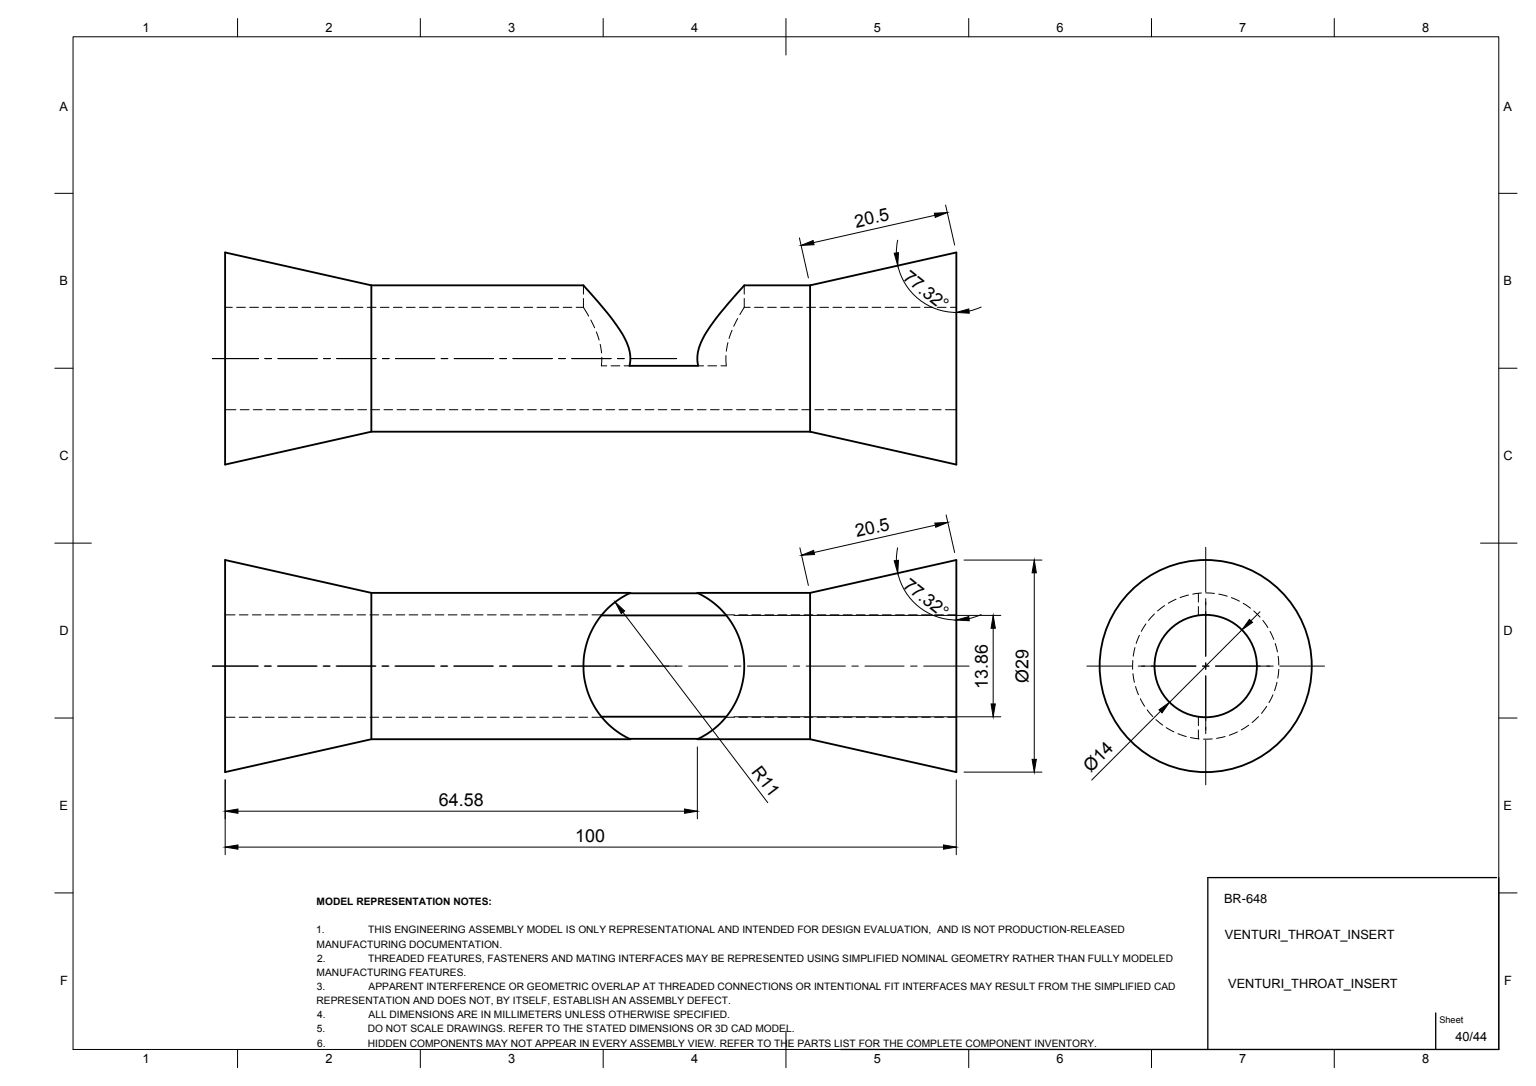
ISO-10303-21;
HEADER;
FILE_DESCRIPTION((''),'2;1');
FILE_NAME('VENTURI_THROAT_INSERT.step','2026-10-01T22:05:39-07:00',(''),(''),'','','');
FILE_SCHEMA (('AUTOMOTIVE_DESIGN { 1 0 10303 214 3 1 1 }'));
ENDSEC;
DATA;
#10=MECHANICAL_DESIGN_GEOMETRIC_PRESENTATION_REPRESENTATION('',(#636),#24628);
#11=CONICAL_SURFACE('',#15204,1.225,0.221314442347791) ;
#12=CONICAL_SURFACE('',#15210,1.225,0.221314442347791) ;
#552=SHAPE_REPRESENTATION_RELATIONSHIP('SRR','None',#24826,#594) ;
#594=ADVANCED_BREP_SHAPE_REPRESENTATION('',(#675),#24616) ;
#636=STYLED_ITEM('',(#25035),#675) ;
#675=MANIFOLD_SOLID_BREP('VENTURI_THROAT_INSERT',#13178) ;
#910=FACE_BOUND('',#4625,.T.) ;
#911=FACE_BOUND('',#4629,.T.) ;
#991=B_SPLINE_CURVE_WITH_KNOTS('',3,(#23937,#23938,#23939,#23940,#23941,
#23942,#23943,#23944,#23945,#23946,#23947,#23948,#23949),.UNSPECIFIED.,
 .F.,.F.,(4,3,2,2,2,4),(-0.0993179449412329,0.,0.274566149486996,0.549132298973992,
0.821321935999811,1.09351157302563),.UNSPECIFIED.) ;
#992=B_SPLINE_CURVE_WITH_KNOTS('',3,(#23951,#23952,#23953,#23954,#23955,
#23956,#23957,#23958,#23959,#23960,#23961,#23962,#23963,#23964,#23965,#23966,
#23967),.UNSPECIFIED.,.F.,.F.,(4,2,2,2,2,2,3,4),(-1.69011593432845,-1.48746936798106,
-1.28482280163367,-0.87952966893888,-0.43976483446944,-0.219882417234721,
0.,0.10342060321835),.UNSPECIFIED.) ;
#993=B_SPLINE_CURVE_WITH_KNOTS('',3,(#23969,#23970,#23971,#23972,#23973,
#23974,#23975,#23976,#23977,#23978,#23979,#23980,#23981,#23982,#23983,#23984),
 .UNSPECIFIED.,.F.,.F.,(4,2,2,2,2,2,2,4),(-3.48365246791255,-3.38023186865691,
-3.16034945142219,-2.94046703418747,-2.50070219971803,-2.09540906702324,
-1.89276250067585,-1.69011593432845),.UNSPECIFIED.) ;
#994=B_SPLINE_CURVE_WITH_KNOTS('',3,(#23987,#23988,#23989,#23990,#23991,
#23992,#23993,#23994,#23995,#23996,#23997,#23998),.UNSPECIFIED.,.F.,.F.,
(4,2,2,2,2,4),(1.09351157302563,1.36570121005145,1.63789084707727,1.91245699656426,
2.18702314605126,2.28634110246251),.UNSPECIFIED.) ;
#995=B_SPLINE_CURVE_WITH_KNOTS('',3,(#24002,#24003,#24004,#24005,#24006,
#24007,#24008,#24009,#24010,#24011,#24012,#24013),.UNSPECIFIED.,.F.,.F.,
(4,2,2,2,2,4),(-2.28634109099249,-2.18702314605126,-1.91245699656426,-1.63789084707727,
-1.36570121005145,-1.09351157302563),.UNSPECIFIED.) ;
#996=B_SPLINE_CURVE_WITH_KNOTS('',3,(#24017,#24018,#24019,#24020,#24021,
#24022,#24023,#24024,#24025,#24026,#24027,#24028,#24029,#24030,#24031,#24032),
 .UNSPECIFIED.,.F.,.F.,(4,2,2,2,2,2,2,4),(1.69011593432845,1.89276250067585,
2.09540906702324,2.50070219971803,2.94046703418747,3.16034945142219,3.38023186865691,
3.48365247187527),.UNSPECIFIED.) ;
#997=B_SPLINE_CURVE_WITH_KNOTS('',3,(#24033,#24034,#24035,#24036,#24037,
#24038,#24039,#24040,#24041,#24042,#24043,#24044,#24045,#24046,#24047,#24048,
#24049),.UNSPECIFIED.,.F.,.F.,(4,3,2,2,2,2,2,4),(-0.103420599255634,0.,
0.21988241723472,0.43976483446944,0.87952966893888,1.28482280163367,1.48746936798106,
1.69011593432845),.UNSPECIFIED.) ;
#998=B_SPLINE_CURVE_WITH_KNOTS('',3,(#24050,#24051,#24052,#24053,#24054,
#24055,#24056,#24057,#24058,#24059,#24060,#24061,#24062),.UNSPECIFIED.,
 .F.,.F.,(4,2,2,2,3,4),(-1.09351157302563,-0.821321935999811,-0.549132298973992,
-0.274566149486996,0.,0.0993179564112534),.UNSPECIFIED.) ;
#1712=LINE('',#23929,#2548) ;
#1713=LINE('',#23933,#2549) ;
#1714=LINE('',#24064,#2550) ;
#1715=LINE('',#24065,#2551) ;
#1716=LINE('',#24069,#2552) ;
#1717=LINE('',#24071,#2553) ;
#1718=LINE('',#24077,#2554) ;
#1719=LINE('',#24081,#2555) ;
#1720=LINE('',#24083,#2556) ;
#1721=LINE('',#24087,#2557) ;
#2548=VECTOR('',#19185,1.) ;
#2549=VECTOR('',#19188,1.) ;
#2550=VECTOR('',#19201,1.) ;
#2551=VECTOR('',#19202,1.) ;
#2552=VECTOR('',#19207,0.7) ;
#2553=VECTOR('',#19208,0.7) ;
#2554=VECTOR('',#19215,1.225) ;
#2555=VECTOR('',#19222,1.) ;
#2556=VECTOR('',#19223,1.) ;
#2557=VECTOR('',#19228,1.225) ;
#2920=CYLINDRICAL_SURFACE('',#15196,1.1) ;
#2921=CYLINDRICAL_SURFACE('',#15198,1.1) ;
#2922=CYLINDRICAL_SURFACE('',#15201,0.7) ;
#2923=CYLINDRICAL_SURFACE('',#15208,1.) ;
#3627=FACE_OUTER_BOUND('',#4618,.T.) ;
#3628=FACE_OUTER_BOUND('',#4619,.T.) ;
#3629=FACE_OUTER_BOUND('',#4620,.T.) ;
#3630=FACE_OUTER_BOUND('',#4621,.T.) ;
#3631=FACE_OUTER_BOUND('',#4622,.T.) ;
#3632=FACE_OUTER_BOUND('',#4623,.T.) ;
#3633=FACE_OUTER_BOUND('',#4624,.T.) ;
#3634=FACE_OUTER_BOUND('',#4626,.T.) ;
#3635=FACE_OUTER_BOUND('',#4627,.T.) ;
#3636=FACE_OUTER_BOUND('',#4628,.T.) ;
#4618=EDGE_LOOP('',(#11597,#11598,#11599,#11600)) ;
#4619=EDGE_LOOP('',(#11601,#11602,#11603,#11604,#11605,#11606)) ;
#4620=EDGE_LOOP('',(#11607,#11608,#11609,#11610,#11611,#11612)) ;
#4621=EDGE_LOOP('',(#11613,#11614,#11615,#11616)) ;
#4622=EDGE_LOOP('',(#11617,#11618,#11619,#11620,#11621,#11622,#11623,#11624,
#11625,#11626,#11627,#11628)) ;
#4623=EDGE_LOOP('',(#11629,#11630,#11631,#11632)) ;
#4624=EDGE_LOOP('',(#11633)) ;
#4625=EDGE_LOOP('',(#11634)) ;
#4626=EDGE_LOOP('',(#11635,#11636,#11637,#11638,#11639,#11640,#11641,#11642,
#11643,#11644,#11645,#11646)) ;
#4627=EDGE_LOOP('',(#11647,#11648,#11649,#11650)) ;
#4628=EDGE_LOOP('',(#11651)) ;
#4629=EDGE_LOOP('',(#11652)) ;
#5473=CIRCLE('',#15194,1.1) ;
#5474=CIRCLE('',#15195,1.1) ;
#5475=CIRCLE('',#15197,1.1) ;
#5476=CIRCLE('',#15199,1.1) ;
#5477=CIRCLE('',#15202,0.7) ;
#5478=CIRCLE('',#15203,0.7) ;
#5479=CIRCLE('',#15205,1.45) ;
#5480=CIRCLE('',#15206,1.) ;
#5481=CIRCLE('',#15209,1.) ;
#5482=CIRCLE('',#15211,1.45) ;
#6601=VERTEX_POINT('',#23927) ;
#6602=VERTEX_POINT('',#23928) ;
#6603=VERTEX_POINT('',#23930) ;
#6604=VERTEX_POINT('',#23932) ;
#6605=VERTEX_POINT('',#23936) ;
#6606=VERTEX_POINT('',#23950) ;
#6607=VERTEX_POINT('',#23968) ;
#6608=VERTEX_POINT('',#23985) ;
#6609=VERTEX_POINT('',#24000) ;
#6610=VERTEX_POINT('',#24001) ;
#6611=VERTEX_POINT('',#24014) ;
#6612=VERTEX_POINT('',#24016) ;
#6613=VERTEX_POINT('',#24067) ;
#6614=VERTEX_POINT('',#24070) ;
#6615=VERTEX_POINT('',#24074) ;
#6616=VERTEX_POINT('',#24076) ;
#6617=VERTEX_POINT('',#24082) ;
#6618=VERTEX_POINT('',#24086) ;
#8288=EDGE_CURVE('',#6601,#6602,#1712,.T.) ;
#8289=EDGE_CURVE('',#6603,#6601,#5473,.T.) ;
#8290=EDGE_CURVE('',#6604,#6603,#1713,.T.) ;
#8291=EDGE_CURVE('',#6602,#6604,#5474,.T.) ;
#8292=EDGE_CURVE('',#6602,#6605,#991,.T.) ;
#8293=EDGE_CURVE('',#6606,#6604,#992,.T.) ;
#8294=EDGE_CURVE('',#6607,#6606,#993,.T.) ;
#8295=EDGE_CURVE('',#6607,#6608,#5475,.T.) ;
#8296=EDGE_CURVE('',#6605,#6608,#994,.T.) ;
#8297=EDGE_CURVE('',#6609,#6610,#995,.T.) ;
#8298=EDGE_CURVE('',#6609,#6611,#5476,.T.) ;
#8299=EDGE_CURVE('',#6612,#6611,#996,.T.) ;
#8300=EDGE_CURVE('',#6603,#6612,#997,.T.) ;
#8301=EDGE_CURVE('',#6610,#6601,#998,.T.) ;
#8302=EDGE_CURVE('',#6608,#6609,#1714,.T.) ;
#8303=EDGE_CURVE('',#6611,#6607,#1715,.T.) ;
#8304=EDGE_CURVE('',#6613,#6613,#5477,.T.) ;
#8305=EDGE_CURVE('',#6613,#6605,#1716,.T.) ;
#8306=EDGE_CURVE('',#6610,#6614,#1717,.T.) ;
#8307=EDGE_CURVE('',#6614,#6614,#5478,.T.) ;
#8308=EDGE_CURVE('',#6615,#6615,#5479,.T.) ;
#8309=EDGE_CURVE('',#6615,#6616,#1718,.T.) ;
#8310=EDGE_CURVE('',#6616,#6616,#5480,.T.) ;
#8311=EDGE_CURVE('',#6616,#6612,#1719,.T.) ;
#8312=EDGE_CURVE('',#6606,#6617,#1720,.T.) ;
#8313=EDGE_CURVE('',#6617,#6617,#5481,.T.) ;
#8314=EDGE_CURVE('',#6617,#6618,#1721,.T.) ;
#8315=EDGE_CURVE('',#6618,#6618,#5482,.T.) ;
#11597=ORIENTED_EDGE('',*,*,#8288,.F.) ;
#11598=ORIENTED_EDGE('',*,*,#8289,.F.) ;
#11599=ORIENTED_EDGE('',*,*,#8290,.F.) ;
#11600=ORIENTED_EDGE('',*,*,#8291,.F.) ;
#11601=ORIENTED_EDGE('',*,*,#8292,.F.) ;
#11602=ORIENTED_EDGE('',*,*,#8291,.T.) ;
#11603=ORIENTED_EDGE('',*,*,#8293,.F.) ;
#11604=ORIENTED_EDGE('',*,*,#8294,.F.) ;
#11605=ORIENTED_EDGE('',*,*,#8295,.T.) ;
#11606=ORIENTED_EDGE('',*,*,#8296,.F.) ;
#11607=ORIENTED_EDGE('',*,*,#8297,.F.) ;
#11608=ORIENTED_EDGE('',*,*,#8298,.T.) ;
#11609=ORIENTED_EDGE('',*,*,#8299,.F.) ;
#11610=ORIENTED_EDGE('',*,*,#8300,.F.) ;
#11611=ORIENTED_EDGE('',*,*,#8289,.T.) ;
#11612=ORIENTED_EDGE('',*,*,#8301,.F.) ;
#11613=ORIENTED_EDGE('',*,*,#8302,.F.) ;
#11614=ORIENTED_EDGE('',*,*,#8295,.F.) ;
#11615=ORIENTED_EDGE('',*,*,#8303,.F.) ;
#11616=ORIENTED_EDGE('',*,*,#8298,.F.) ;
#11617=ORIENTED_EDGE('',*,*,#8304,.F.) ;
#11618=ORIENTED_EDGE('',*,*,#8305,.T.) ;
#11619=ORIENTED_EDGE('',*,*,#8296,.T.) ;
#11620=ORIENTED_EDGE('',*,*,#8302,.T.) ;
#11621=ORIENTED_EDGE('',*,*,#8297,.T.) ;
#11622=ORIENTED_EDGE('',*,*,#8306,.T.) ;
#11623=ORIENTED_EDGE('',*,*,#8307,.F.) ;
#11624=ORIENTED_EDGE('',*,*,#8306,.F.) ;
#11625=ORIENTED_EDGE('',*,*,#8301,.T.) ;
#11626=ORIENTED_EDGE('',*,*,#8288,.T.) ;
#11627=ORIENTED_EDGE('',*,*,#8292,.T.) ;
#11628=ORIENTED_EDGE('',*,*,#8305,.F.) ;
#11629=ORIENTED_EDGE('',*,*,#8308,.F.) ;
#11630=ORIENTED_EDGE('',*,*,#8309,.T.) ;
#11631=ORIENTED_EDGE('',*,*,#8310,.T.) ;
#11632=ORIENTED_EDGE('',*,*,#8309,.F.) ;
#11633=ORIENTED_EDGE('',*,*,#8308,.T.) ;
#11634=ORIENTED_EDGE('',*,*,#8307,.T.) ;
#11635=ORIENTED_EDGE('',*,*,#8310,.F.) ;
#11636=ORIENTED_EDGE('',*,*,#8311,.T.) ;
#11637=ORIENTED_EDGE('',*,*,#8299,.T.) ;
#11638=ORIENTED_EDGE('',*,*,#8303,.T.) ;
#11639=ORIENTED_EDGE('',*,*,#8294,.T.) ;
#11640=ORIENTED_EDGE('',*,*,#8312,.T.) ;
#11641=ORIENTED_EDGE('',*,*,#8313,.T.) ;
#11642=ORIENTED_EDGE('',*,*,#8312,.F.) ;
#11643=ORIENTED_EDGE('',*,*,#8293,.T.) ;
#11644=ORIENTED_EDGE('',*,*,#8290,.T.) ;
#11645=ORIENTED_EDGE('',*,*,#8300,.T.) ;
#11646=ORIENTED_EDGE('',*,*,#8311,.F.) ;
#11647=ORIENTED_EDGE('',*,*,#8313,.F.) ;
#11648=ORIENTED_EDGE('',*,*,#8314,.T.) ;
#11649=ORIENTED_EDGE('',*,*,#8315,.F.) ;
#11650=ORIENTED_EDGE('',*,*,#8314,.F.) ;
#11651=ORIENTED_EDGE('',*,*,#8315,.T.) ;
#11652=ORIENTED_EDGE('',*,*,#8304,.T.) ;
#12289=PLANE('',#15193) ;
#12290=PLANE('',#15200) ;
#12291=PLANE('',#15207) ;
#12292=PLANE('',#15212) ;
#13022=ADVANCED_FACE('',(#3627),#12289,.F.) ;
#13023=ADVANCED_FACE('',(#3628),#2920,.F.) ;
#13024=ADVANCED_FACE('',(#3629),#2921,.F.) ;
#13025=ADVANCED_FACE('',(#3630),#12290,.F.) ;
#13026=ADVANCED_FACE('',(#3631),#2922,.F.) ;
#13027=ADVANCED_FACE('',(#3632),#11,.T.) ;
#13028=ADVANCED_FACE('',(#3633,#910),#12291,.T.) ;
#13029=ADVANCED_FACE('',(#3634),#2923,.T.) ;
#13030=ADVANCED_FACE('',(#3635),#12,.T.) ;
#13031=ADVANCED_FACE('',(#3636,#911),#12292,.T.) ;
#13178=CLOSED_SHELL('',(#13022,#13023,#13024,#13025,#13026,#13027,#13028,
#13029,#13030,#13031)) ;
#15192=AXIS2_PLACEMENT_3D('',#23925,#19181,#19182) ;
#15193=AXIS2_PLACEMENT_3D('',#23926,#19183,#19184) ;
#15194=AXIS2_PLACEMENT_3D('',#23931,#19186,#19187) ;
#15195=AXIS2_PLACEMENT_3D('',#23934,#19189,#19190) ;
#15196=AXIS2_PLACEMENT_3D('',#23935,#19191,#19192) ;
#15197=AXIS2_PLACEMENT_3D('',#23986,#19193,#19194) ;
#15198=AXIS2_PLACEMENT_3D('',#23999,#19195,#19196) ;
#15199=AXIS2_PLACEMENT_3D('',#24015,#19197,#19198) ;
#15200=AXIS2_PLACEMENT_3D('',#24063,#19199,#19200) ;
#15201=AXIS2_PLACEMENT_3D('',#24066,#19203,#19204) ;
#15202=AXIS2_PLACEMENT_3D('',#24068,#19205,#19206) ;
#15203=AXIS2_PLACEMENT_3D('',#24072,#19209,#19210) ;
#15204=AXIS2_PLACEMENT_3D('',#24073,#19211,#19212) ;
#15205=AXIS2_PLACEMENT_3D('',#24075,#19213,#19214) ;
#15206=AXIS2_PLACEMENT_3D('',#24078,#19216,#19217) ;
#15207=AXIS2_PLACEMENT_3D('',#24079,#19218,#19219) ;
#15208=AXIS2_PLACEMENT_3D('',#24080,#19220,#19221) ;
#15209=AXIS2_PLACEMENT_3D('',#24084,#19224,#19225) ;
#15210=AXIS2_PLACEMENT_3D('',#24085,#19226,#19227) ;
#15211=AXIS2_PLACEMENT_3D('',#24088,#19229,#19230) ;
#15212=AXIS2_PLACEMENT_3D('',#24089,#19231,#19232) ;
#19181=DIRECTION('axis',(0.,0.,1.)) ;
#19182=DIRECTION('refdir',(1.,0.,0.)) ;
#19183=DIRECTION('center_axis',(0.,0.,-1.)) ;
#19184=DIRECTION('ref_axis',(-1.,0.,0.)) ;
#19185=DIRECTION('',(-1.,0.,0.)) ;
#19186=DIRECTION('center_axis',(0.,0.,-1.)) ;
#19187=DIRECTION('ref_axis',(1.,0.,0.)) ;
#19188=DIRECTION('',(1.,0.,0.)) ;
#19189=DIRECTION('center_axis',(0.,0.,-1.)) ;
#19190=DIRECTION('ref_axis',(1.,0.,0.)) ;
#19191=DIRECTION('center_axis',(0.,0.,1.)) ;
#19192=DIRECTION('ref_axis',(-1.,-1.22464679914735E-16,0.)) ;
#19193=DIRECTION('center_axis',(0.,0.,-1.)) ;
#19194=DIRECTION('ref_axis',(1.,0.,0.)) ;
#19195=DIRECTION('center_axis',(0.,0.,1.)) ;
#19196=DIRECTION('ref_axis',(1.,0.,0.)) ;
#19197=DIRECTION('center_axis',(0.,0.,-1.)) ;
#19198=DIRECTION('ref_axis',(1.,0.,0.)) ;
#19199=DIRECTION('center_axis',(0.,0.,-1.)) ;
#19200=DIRECTION('ref_axis',(-1.,0.,0.)) ;
#19201=DIRECTION('',(1.,0.,0.)) ;
#19202=DIRECTION('',(-1.,0.,0.)) ;
#19203=DIRECTION('center_axis',(1.,0.,0.)) ;
#19204=DIRECTION('ref_axis',(0.,0.,-1.)) ;
#19205=DIRECTION('center_axis',(1.,0.,0.)) ;
#19206=DIRECTION('ref_axis',(0.,0.,-1.)) ;
#19207=DIRECTION('',(1.,0.,0.)) ;
#19208=DIRECTION('',(1.,0.,0.)) ;
#19209=DIRECTION('center_axis',(-1.,0.,0.)) ;
#19210=DIRECTION('ref_axis',(0.,0.,-1.)) ;
#19211=DIRECTION('center_axis',(1.,0.,0.)) ;
#19212=DIRECTION('ref_axis',(0.,0.,-1.)) ;
#19213=DIRECTION('center_axis',(1.,0.,0.)) ;
#19214=DIRECTION('ref_axis',(0.,0.,-1.)) ;
#19215=DIRECTION('',(-0.975609756097561,2.68824907129907E-17,-0.219512195121951)) ;
#19216=DIRECTION('center_axis',(1.,0.,0.)) ;
#19217=DIRECTION('ref_axis',(0.,0.,-1.)) ;
#19218=DIRECTION('center_axis',(1.,0.,0.)) ;
#19219=DIRECTION('ref_axis',(0.,0.,-1.)) ;
#19220=DIRECTION('center_axis',(1.,0.,0.)) ;
#19221=DIRECTION('ref_axis',(0.,0.,-1.)) ;
#19222=DIRECTION('',(-1.,0.,0.)) ;
#19223=DIRECTION('',(-1.,0.,0.)) ;
#19224=DIRECTION('center_axis',(1.,0.,0.)) ;
#19225=DIRECTION('ref_axis',(0.,0.,-1.)) ;
#19226=DIRECTION('center_axis',(-1.,0.,0.)) ;
#19227=DIRECTION('ref_axis',(0.,0.,-1.)) ;
#19228=DIRECTION('',(-0.975609756097561,-2.68824907129907E-17,0.219512195121951)) ;
#19229=DIRECTION('center_axis',(-1.,0.,0.)) ;
#19230=DIRECTION('ref_axis',(0.,0.,-1.)) ;
#19231=DIRECTION('center_axis',(-1.,0.,0.)) ;
#19232=DIRECTION('ref_axis',(0.,0.,1.)) ;
#23925=CARTESIAN_POINT('',(0.,0.,0.)) ;
#23926=CARTESIAN_POINT('Origin',(-3.,-1.8,-16.6)) ;
#23927=CARTESIAN_POINT('',(-2.14559962546825,-1.10717967697245,-16.6)) ;
#23928=CARTESIAN_POINT('',(-3.85440037453175,-1.10717967697245,-16.6)) ;
#23929=CARTESIAN_POINT('',(-4.,-1.10717967697245,-16.6)) ;
#23930=CARTESIAN_POINT('',(-2.53095842401766,-0.80501256289338,-16.6)) ;
#23931=CARTESIAN_POINT('Origin',(-3.,-1.8,-16.6)) ;
#23932=CARTESIAN_POINT('',(-3.46904157598234,-0.80501256289338,-16.6)) ;
#23933=CARTESIAN_POINT('',(-4.,-0.80501256289338,-16.6)) ;
#23934=CARTESIAN_POINT('Origin',(-3.,-1.8,-16.6)) ;
#23935=CARTESIAN_POINT('Origin',(-3.,-1.8,-15.55)) ;
#23936=CARTESIAN_POINT('',(-4.1,-1.8,-15.8)) ;
#23937=CARTESIAN_POINT('Ctrl Pts',(-3.85440037453175,-1.10717967697245,
-16.6)) ;
#23938=CARTESIAN_POINT('Ctrl Pts',(-3.85049705318298,-1.10236602022558,
-16.5666500077769)) ;
#23939=CARTESIAN_POINT('Ctrl Pts',(-3.84852813742386,-1.1,-16.5331059816471)) ;
#23940=CARTESIAN_POINT('Ctrl Pts',(-3.84852813742386,-1.1,-16.5)) ;
#23941=CARTESIAN_POINT('Ctrl Pts',(-3.84852813742386,-1.1,-16.408477950171)) ;
#23942=CARTESIAN_POINT('Ctrl Pts',(-3.86487430708359,-1.11884674360792,
-16.3138744868034)) ;
#23943=CARTESIAN_POINT('Ctrl Pts',(-3.91703156085527,-1.19087751926739,
-16.1428129676115)) ;
#23944=CARTESIAN_POINT('Ctrl Pts',(-3.95162711030062,-1.24406317485413,
-16.0659873314847)) ;
#23945=CARTESIAN_POINT('Ctrl Pts',(-4.01279528835241,-1.36545967307144,
-15.9445908332674)) ;
#23946=CARTESIAN_POINT('Ctrl Pts',(-4.04402775497001,-1.44241519978942,
-15.8910472783858)) ;
#23947=CARTESIAN_POINT('Ctrl Pts',(-4.08782165352582,-1.6142450358863,-15.8186884461636)) ;
#23948=CARTESIAN_POINT('Ctrl Pts',(-4.1,-1.70927012099139,-15.8)) ;
#23949=CARTESIAN_POINT('Ctrl Pts',(-4.1,-1.8,-15.8)) ;
#23950=CARTESIAN_POINT('',(-4.1,-1.8,-15.5)) ;
#23951=CARTESIAN_POINT('Ctrl Pts',(-4.1,-1.8,-15.5)) ;
#23952=CARTESIAN_POINT('Ctrl Pts',(-4.1,-1.73245114455087,-15.5)) ;
#23953=CARTESIAN_POINT('Ctrl Pts',(-4.09366900622909,-1.66396811523288,
-15.5069510256229)) ;
#23954=CARTESIAN_POINT('Ctrl Pts',(-4.06861417966391,-1.53040715178794,
-15.5346137377671)) ;
#23955=CARTESIAN_POINT('Ctrl Pts',(-4.04990213252851,-1.46532446507313,
-15.5553131496202)) ;
#23956=CARTESIAN_POINT('Ctrl Pts',(-3.97908681363415,-1.28173592783325,
-15.6344562293198)) ;
#23957=CARTESIAN_POINT('Ctrl Pts',(-3.91155673921738,-1.17504680959349,
-15.7107396280334)) ;
#23958=CARTESIAN_POINT('Ctrl Pts',(-3.76780945986836,-1.00375215686099,
-15.8820342807659)) ;
#23959=CARTESIAN_POINT('Ctrl Pts',(-3.67938152899323,-0.930008802100376,
-15.9904145776246)) ;
#23960=CARTESIAN_POINT('Ctrl Pts',(-3.56405332421194,-0.85450777858214,
-16.1680616160286)) ;
#23961=CARTESIAN_POINT('Ctrl Pts',(-3.52879854306256,-0.834982894950926,
-16.2296167208294)) ;
#23962=CARTESIAN_POINT('Ctrl Pts',(-3.47583842827067,-0.807798528642412,
-16.3589280031455)) ;
#23963=CARTESIAN_POINT('Ctrl Pts',(-3.45825756949558,-0.8,-16.4267058609218)) ;
#23964=CARTESIAN_POINT('Ctrl Pts',(-3.45825756949558,-0.8,-16.5)) ;
#23965=CARTESIAN_POINT('Ctrl Pts',(-3.45825756949558,-0.8,-16.5344735344061)) ;
#23966=CARTESIAN_POINT('Ctrl Pts',(-3.46215940235726,-0.801768275133648,
-16.5677197443671)) ;
#23967=CARTESIAN_POINT('Ctrl Pts',(-3.46904157598234,-0.80501256289338,
-16.6)) ;
#23968=CARTESIAN_POINT('',(-3.46904157598234,-2.79498743710662,-16.6)) ;
#23969=CARTESIAN_POINT('Ctrl Pts',(-3.46904157598234,-2.79498743710662,
-16.6)) ;
#23970=CARTESIAN_POINT('Ctrl Pts',(-3.46215940232543,-2.79823172488136,
-16.5677197442178)) ;
#23971=CARTESIAN_POINT('Ctrl Pts',(-3.45825756949559,-2.8,-16.5344735330852)) ;
#23972=CARTESIAN_POINT('Ctrl Pts',(-3.45825756949558,-2.8,-16.4267058609218)) ;
#23973=CARTESIAN_POINT('Ctrl Pts',(-3.47583842827066,-2.79220147135759,
-16.3589280031455)) ;
#23974=CARTESIAN_POINT('Ctrl Pts',(-3.52879854306256,-2.76501710504908,
-16.2296167208294)) ;
#23975=CARTESIAN_POINT('Ctrl Pts',(-3.56405332421193,-2.74549222141786,
-16.1680616160286)) ;
#23976=CARTESIAN_POINT('Ctrl Pts',(-3.67938152899323,-2.66999119789963,
-15.9904145776246)) ;
#23977=CARTESIAN_POINT('Ctrl Pts',(-3.76780945986836,-2.59624784313901,
-15.8820342807659)) ;
#23978=CARTESIAN_POINT('Ctrl Pts',(-3.91155673921738,-2.42495319040651,
-15.7107396280334)) ;
#23979=CARTESIAN_POINT('Ctrl Pts',(-3.97908681363414,-2.31826407216675,
-15.6344562293198)) ;
#23980=CARTESIAN_POINT('Ctrl Pts',(-4.04990213252851,-2.13467553492687,
-15.5553131496202)) ;
#23981=CARTESIAN_POINT('Ctrl Pts',(-4.06861417966391,-2.06959284821206,
-15.5346137377671)) ;
#23982=CARTESIAN_POINT('Ctrl Pts',(-4.09366900622909,-1.93603188476712,
-15.5069510256229)) ;
#23983=CARTESIAN_POINT('Ctrl Pts',(-4.1,-1.86754885544913,-15.5)) ;
#23984=CARTESIAN_POINT('Ctrl Pts',(-4.1,-1.8,-15.5)) ;
#23985=CARTESIAN_POINT('',(-3.85440037453175,-2.49282032302755,-16.6)) ;
#23986=CARTESIAN_POINT('Origin',(-3.,-1.8,-16.6)) ;
#23987=CARTESIAN_POINT('Ctrl Pts',(-4.1,-1.8,-15.8)) ;
#23988=CARTESIAN_POINT('Ctrl Pts',(-4.1,-1.89072987900861,-15.8)) ;
#23989=CARTESIAN_POINT('Ctrl Pts',(-4.08782165352582,-1.9857549641137,-15.8186884461636)) ;
#23990=CARTESIAN_POINT('Ctrl Pts',(-4.04402775497001,-2.15758480021059,
-15.8910472783858)) ;
#23991=CARTESIAN_POINT('Ctrl Pts',(-4.01279528835241,-2.23454032692856,
-15.9445908332674)) ;
#23992=CARTESIAN_POINT('Ctrl Pts',(-3.95162711030062,-2.35593682514587,
-16.0659873314847)) ;
#23993=CARTESIAN_POINT('Ctrl Pts',(-3.91703156085527,-2.40912248073261,
-16.1428129676115)) ;
#23994=CARTESIAN_POINT('Ctrl Pts',(-3.86487430708359,-2.48115325639208,
-16.3138744868034)) ;
#23995=CARTESIAN_POINT('Ctrl Pts',(-3.84852813742386,-2.5,-16.408477950171)) ;
#23996=CARTESIAN_POINT('Ctrl Pts',(-3.84852813742386,-2.5,-16.5331059854704)) ;
#23997=CARTESIAN_POINT('Ctrl Pts',(-3.85049705337729,-2.4976339795348,-16.5666500094371)) ;
#23998=CARTESIAN_POINT('Ctrl Pts',(-3.85440037453175,-2.49282032302755,
-16.6)) ;
#23999=CARTESIAN_POINT('Origin',(-3.,-1.8,-15.55)) ;
#24000=CARTESIAN_POINT('',(-2.14559962546825,-2.49282032302755,-16.6)) ;
#24001=CARTESIAN_POINT('',(-1.9,-1.8,-15.8)) ;
#24002=CARTESIAN_POINT('Ctrl Pts',(-2.14559962546825,-2.49282032302755,
-16.6)) ;
#24003=CARTESIAN_POINT('Ctrl Pts',(-2.14950294681702,-2.49763397977442,
-16.5666500077769)) ;
#24004=CARTESIAN_POINT('Ctrl Pts',(-2.15147186257614,-2.5,-16.5331059816471)) ;
#24005=CARTESIAN_POINT('Ctrl Pts',(-2.15147186257614,-2.5,-16.408477950171)) ;
#24006=CARTESIAN_POINT('Ctrl Pts',(-2.13512569291641,-2.48115325639208,
-16.3138744868034)) ;
#24007=CARTESIAN_POINT('Ctrl Pts',(-2.08296843914473,-2.40912248073261,
-16.1428129676115)) ;
#24008=CARTESIAN_POINT('Ctrl Pts',(-2.04837288969938,-2.35593682514587,
-16.0659873314847)) ;
#24009=CARTESIAN_POINT('Ctrl Pts',(-1.98720471164759,-2.23454032692856,
-15.9445908332674)) ;
#24010=CARTESIAN_POINT('Ctrl Pts',(-1.95597224502999,-2.15758480021059,
-15.8910472783858)) ;
#24011=CARTESIAN_POINT('Ctrl Pts',(-1.91217834647418,-1.9857549641137,-15.8186884461636)) ;
#24012=CARTESIAN_POINT('Ctrl Pts',(-1.9,-1.89072987900861,-15.8)) ;
#24013=CARTESIAN_POINT('Ctrl Pts',(-1.9,-1.8,-15.8)) ;
#24014=CARTESIAN_POINT('',(-2.53095842401766,-2.79498743710662,-16.6)) ;
#24015=CARTESIAN_POINT('Origin',(-3.,-1.8,-16.6)) ;
#24016=CARTESIAN_POINT('',(-1.9,-1.8,-15.5)) ;
#24017=CARTESIAN_POINT('Ctrl Pts',(-1.9,-1.8,-15.5)) ;
#24018=CARTESIAN_POINT('Ctrl Pts',(-1.9,-1.86754885544913,-15.5)) ;
#24019=CARTESIAN_POINT('Ctrl Pts',(-1.90633099377091,-1.93603188476712,
-15.5069510256229)) ;
#24020=CARTESIAN_POINT('Ctrl Pts',(-1.93138582033609,-2.06959284821206,
-15.5346137377671)) ;
#24021=CARTESIAN_POINT('Ctrl Pts',(-1.95009786747149,-2.13467553492686,
-15.5553131496202)) ;
#24022=CARTESIAN_POINT('Ctrl Pts',(-2.02091318636585,-2.31826407216675,
-15.6344562293198)) ;
#24023=CARTESIAN_POINT('Ctrl Pts',(-2.08844326078262,-2.42495319040651,
-15.7107396280334)) ;
#24024=CARTESIAN_POINT('Ctrl Pts',(-2.23219054013164,-2.59624784313901,
-15.8820342807659)) ;
#24025=CARTESIAN_POINT('Ctrl Pts',(-2.32061847100677,-2.66999119789963,
-15.9904145776246)) ;
#24026=CARTESIAN_POINT('Ctrl Pts',(-2.43594667578807,-2.74549222141786,
-16.1680616160286)) ;
#24027=CARTESIAN_POINT('Ctrl Pts',(-2.47120145693744,-2.76501710504908,
-16.2296167208294)) ;
#24028=CARTESIAN_POINT('Ctrl Pts',(-2.52416157172934,-2.79220147135759,
-16.3589280031455)) ;
#24029=CARTESIAN_POINT('Ctrl Pts',(-2.54174243050442,-2.8,-16.4267058609218)) ;
#24030=CARTESIAN_POINT('Ctrl Pts',(-2.54174243050442,-2.8,-16.5344735344061)) ;
#24031=CARTESIAN_POINT('Ctrl Pts',(-2.53784059764274,-2.79823172486635,
-16.5677197443671)) ;
#24032=CARTESIAN_POINT('Ctrl Pts',(-2.53095842401766,-2.79498743710662,
-16.6)) ;
#24033=CARTESIAN_POINT('Ctrl Pts',(-2.53095842401766,-0.80501256289338,
-16.6)) ;
#24034=CARTESIAN_POINT('Ctrl Pts',(-2.53784059767457,-0.801768275118644,
-16.5677197442178)) ;
#24035=CARTESIAN_POINT('Ctrl Pts',(-2.54174243050442,-0.8,-16.5344735330852)) ;
#24036=CARTESIAN_POINT('Ctrl Pts',(-2.54174243050442,-0.8,-16.5)) ;
#24037=CARTESIAN_POINT('Ctrl Pts',(-2.54174243050442,-0.8,-16.4267058609218)) ;
#24038=CARTESIAN_POINT('Ctrl Pts',(-2.52416157172934,-0.807798528642411,
-16.3589280031455)) ;
#24039=CARTESIAN_POINT('Ctrl Pts',(-2.47120145693744,-0.834982894950924,
-16.2296167208294)) ;
#24040=CARTESIAN_POINT('Ctrl Pts',(-2.43594667578807,-0.854507778582139,
-16.1680616160286)) ;
#24041=CARTESIAN_POINT('Ctrl Pts',(-2.32061847100677,-0.930008802100373,
-15.9904145776246)) ;
#24042=CARTESIAN_POINT('Ctrl Pts',(-2.23219054013164,-1.00375215686099,
-15.8820342807659)) ;
#24043=CARTESIAN_POINT('Ctrl Pts',(-2.08844326078262,-1.17504680959349,
-15.7107396280334)) ;
#24044=CARTESIAN_POINT('Ctrl Pts',(-2.02091318636585,-1.28173592783325,
-15.6344562293198)) ;
#24045=CARTESIAN_POINT('Ctrl Pts',(-1.95009786747149,-1.46532446507313,
-15.5553131496202)) ;
#24046=CARTESIAN_POINT('Ctrl Pts',(-1.93138582033609,-1.53040715178794,
-15.5346137377671)) ;
#24047=CARTESIAN_POINT('Ctrl Pts',(-1.90633099377091,-1.66396811523288,
-15.5069510256229)) ;
#24048=CARTESIAN_POINT('Ctrl Pts',(-1.9,-1.73245114455087,-15.5)) ;
#24049=CARTESIAN_POINT('Ctrl Pts',(-1.9,-1.8,-15.5)) ;
#24050=CARTESIAN_POINT('Ctrl Pts',(-1.9,-1.8,-15.8)) ;
#24051=CARTESIAN_POINT('Ctrl Pts',(-1.9,-1.70927012099139,-15.8)) ;
#24052=CARTESIAN_POINT('Ctrl Pts',(-1.91217834647418,-1.6142450358863,-15.8186884461636)) ;
#24053=CARTESIAN_POINT('Ctrl Pts',(-1.95597224502999,-1.44241519978941,
-15.8910472783858)) ;
#24054=CARTESIAN_POINT('Ctrl Pts',(-1.98720471164759,-1.36545967307144,
-15.9445908332674)) ;
#24055=CARTESIAN_POINT('Ctrl Pts',(-2.04837288969938,-1.24406317485413,
-16.0659873314847)) ;
#24056=CARTESIAN_POINT('Ctrl Pts',(-2.08296843914473,-1.19087751926739,
-16.1428129676115)) ;
#24057=CARTESIAN_POINT('Ctrl Pts',(-2.13512569291641,-1.11884674360792,
-16.3138744868034)) ;
#24058=CARTESIAN_POINT('Ctrl Pts',(-2.15147186257614,-1.1,-16.408477950171)) ;
#24059=CARTESIAN_POINT('Ctrl Pts',(-2.15147186257614,-1.1,-16.5)) ;
#24060=CARTESIAN_POINT('Ctrl Pts',(-2.15147186257614,-1.1,-16.5331059854704)) ;
#24061=CARTESIAN_POINT('Ctrl Pts',(-2.14950294662271,-1.1023660204652,-16.5666500094371)) ;
#24062=CARTESIAN_POINT('Ctrl Pts',(-2.14559962546825,-1.10717967697245,
-16.6)) ;
#24063=CARTESIAN_POINT('Origin',(-3.,-1.8,-16.6)) ;
#24064=CARTESIAN_POINT('',(-4.,-2.49282032302755,-16.6)) ;
#24065=CARTESIAN_POINT('',(-4.,-2.79498743710662,-16.6)) ;
#24066=CARTESIAN_POINT('Origin',(-4.,-1.8,-16.5)) ;
#24067=CARTESIAN_POINT('',(-9.,-1.8,-15.8)) ;
#24068=CARTESIAN_POINT('Origin',(-9.,-1.8,-16.5)) ;
#24069=CARTESIAN_POINT('',(-4.,-1.8,-15.8)) ;
#24070=CARTESIAN_POINT('',(1.,-1.8,-15.8)) ;
#24071=CARTESIAN_POINT('',(-4.,-1.8,-15.8)) ;
#24072=CARTESIAN_POINT('Origin',(1.,-1.8,-16.5)) ;
#24073=CARTESIAN_POINT('Origin',(0.,-1.8,-16.5)) ;
#24074=CARTESIAN_POINT('',(1.,-1.8,-15.05)) ;
#24075=CARTESIAN_POINT('Origin',(1.,-1.8,-16.5)) ;
#24076=CARTESIAN_POINT('',(-1.,-1.8,-15.5)) ;
#24077=CARTESIAN_POINT('',(0.,-1.8,-15.275)) ;
#24078=CARTESIAN_POINT('Origin',(-1.,-1.8,-16.5)) ;
#24079=CARTESIAN_POINT('Origin',(1.,-1.8,-16.5)) ;
#24080=CARTESIAN_POINT('Origin',(-4.,-1.8,-16.5)) ;
#24081=CARTESIAN_POINT('',(-4.,-1.8,-15.5)) ;
#24082=CARTESIAN_POINT('',(-7.,-1.8,-15.5)) ;
#24083=CARTESIAN_POINT('',(-4.,-1.8,-15.5)) ;
#24084=CARTESIAN_POINT('Origin',(-7.,-1.8,-16.5)) ;
#24085=CARTESIAN_POINT('Origin',(-8.,-1.8,-16.5)) ;
#24086=CARTESIAN_POINT('',(-9.,-1.8,-15.05)) ;
#24087=CARTESIAN_POINT('',(-8.,-1.8,-15.275)) ;
#24088=CARTESIAN_POINT('Origin',(-9.,-1.8,-16.5)) ;
#24089=CARTESIAN_POINT('Origin',(-9.,-1.8,-16.5)) ;
#24568=UNCERTAINTY_MEASURE_WITH_UNIT(LENGTH_MEASURE(0.001),#24629,
'DISTANCE_ACCURACY_VALUE',
'Maximum model space distance between geometric entities at asserted c
onnectivities') ;
#24580=UNCERTAINTY_MEASURE_WITH_UNIT(LENGTH_MEASURE(0.001),#24629,
'DISTANCE_ACCURACY_VALUE',
'Maximum model space distance between geometric entities at asserted c
onnectivities') ;
#24616=(
GEOMETRIC_REPRESENTATION_CONTEXT(3)
GLOBAL_UNCERTAINTY_ASSIGNED_CONTEXT((#24568))
GLOBAL_UNIT_ASSIGNED_CONTEXT((#24629,#24631,#24632))
REPRESENTATION_CONTEXT('','3D')
) ;
#24628=(
GEOMETRIC_REPRESENTATION_CONTEXT(3)
GLOBAL_UNCERTAINTY_ASSIGNED_CONTEXT((#24580))
GLOBAL_UNIT_ASSIGNED_CONTEXT((#24629,#24631,#24632))
REPRESENTATION_CONTEXT('','3D')
) ;
#24629=(
LENGTH_UNIT()
NAMED_UNIT(*)
SI_UNIT(.CENTI.,.METRE.)
) ;
#24631=(
NAMED_UNIT(*)
PLANE_ANGLE_UNIT()
SI_UNIT($,.RADIAN.)
) ;
#24632=(
NAMED_UNIT(*)
SI_UNIT($,.STERADIAN.)
SOLID_ANGLE_UNIT()
) ;
#24668=SHAPE_DEFINITION_REPRESENTATION(#24749,#24826) ;
#24749=PRODUCT_DEFINITION_SHAPE('',$,#24874) ;
#24826=SHAPE_REPRESENTATION('',(#15192),#24616) ;
#24838=PRODUCT_DEFINITION_CONTEXT('part definition',#24981,'design') ;
#24874=PRODUCT_DEFINITION('VENTURI_THROAT_INSERT',
'VENTURI_THROAT_INSERT',#24921,#24838) ;
#24921=PRODUCT_DEFINITION_FORMATION('',$,#25018) ;
#24981=APPLICATION_CONTEXT(
'Core Data for Automotive Mechanical Design Process') ;
#24982=PRODUCT_CONTEXT('part definition',#24981,'mechanical') ;
#25018=PRODUCT('VENTURI_THROAT_INSERT','VENTURI_THROAT_INSERT',$,(#24982)) ;
#25035=PRESENTATION_STYLE_ASSIGNMENT((#25045)) ;
#25045=SURFACE_STYLE_USAGE(.BOTH.,#25055) ;
#25055=SURFACE_SIDE_STYLE('',(#25065)) ;
#25065=SURFACE_STYLE_FILL_AREA(#25075) ;
#25075=FILL_AREA_STYLE('ABS (White)',(#25085)) ;
#25085=FILL_AREA_STYLE_COLOUR('ABS (White)',#25095) ;
#25095=COLOUR_RGB('ABS (White)', 0.66274510, 0.83137255, 0.94901961) ;
ENDSEC;
END-ISO-10303-21;
